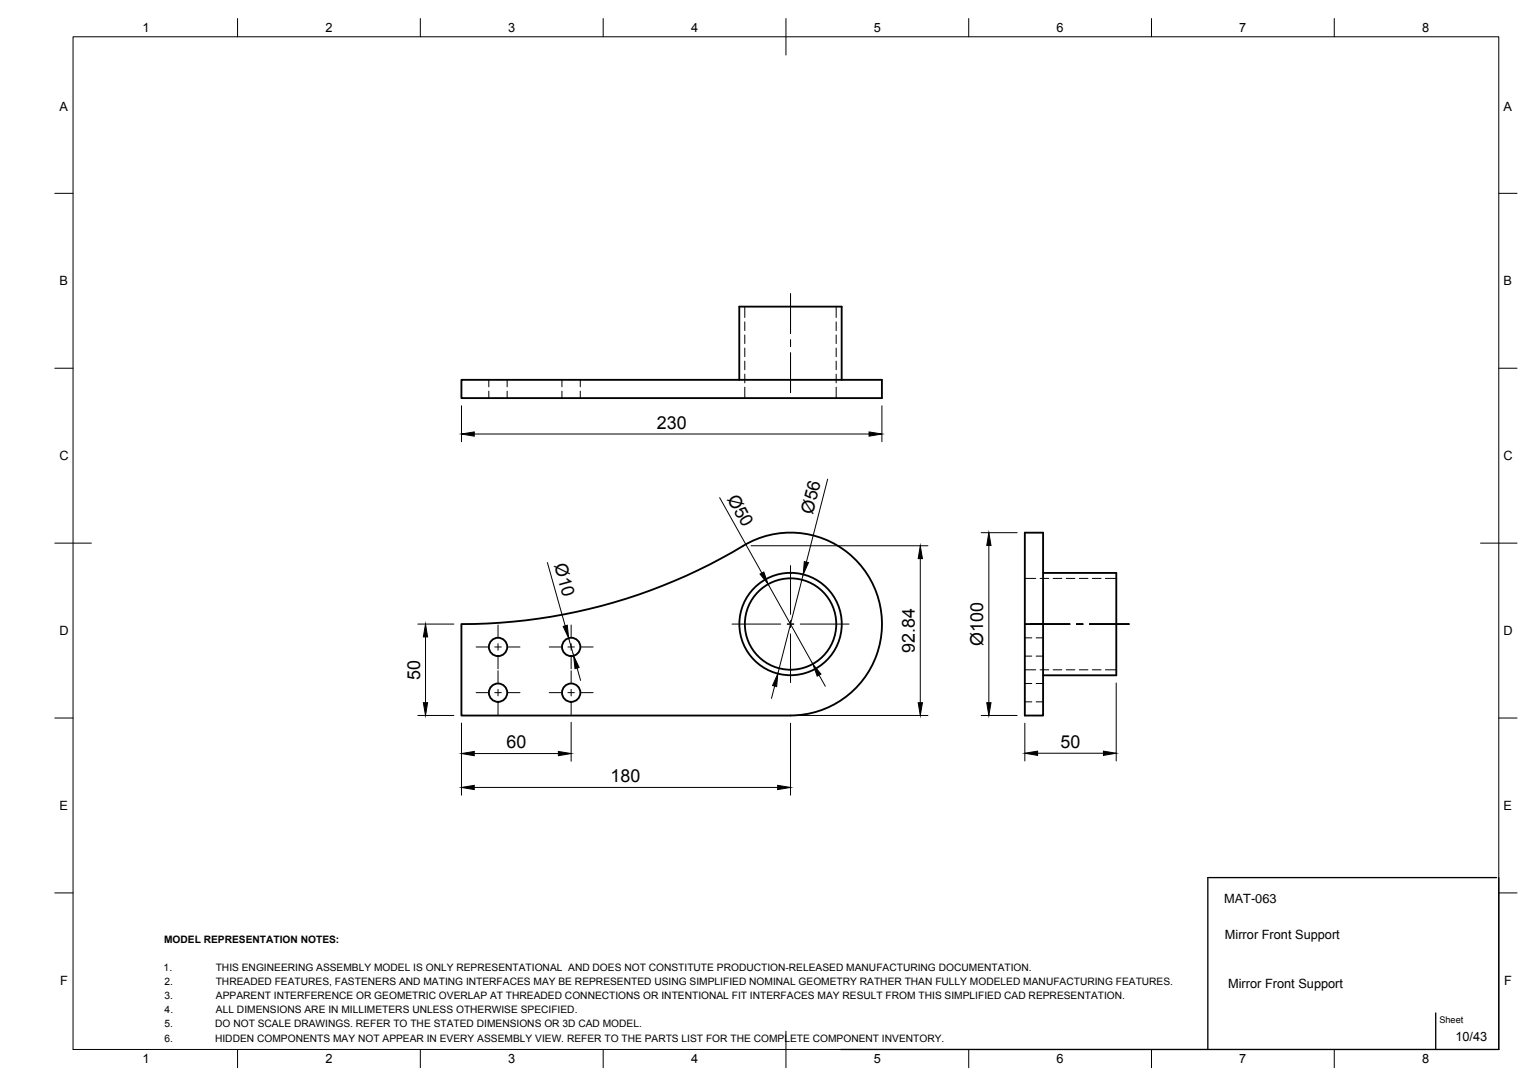
ISO-10303-21;
HEADER;
/* Generated by software containing ST-Developer
 * from STEP Tools, Inc. (www.steptools.com) 
 */

FILE_DESCRIPTION(
/* description */ (''),
/* implementation_level */ '2;1');

FILE_NAME(
/* name */ 'Mirror Front Support.step',
/* time_stamp */ '2026-10-24T09:43:01-07:00',
/* author */ (''),
/* organization */ (''),
/* preprocessor_version */ 'ST-DEVELOPER v20.2',
/* originating_system */ 'Autodesk Translation Framework v15.15.0.0',
/* authorisation */ '');

FILE_SCHEMA (('AUTOMOTIVE_DESIGN { 1 0 10303 214 3 1 1 }'));
ENDSEC;

DATA;
#10=MECHANICAL_DESIGN_GEOMETRIC_PRESENTATION_REPRESENTATION('',(#280),#11112);
#214=SHAPE_REPRESENTATION_RELATIONSHIP('SRR','None',#11237,#247);
#247=ADVANCED_BREP_SHAPE_REPRESENTATION('',(#313),#11082);
#280=STYLED_ITEM('',(#11426),#313);
#313=MANIFOLD_SOLID_BREP('Mirror Front Support',#6017);
#397=FACE_BOUND('',#1228,.T.);
#398=FACE_BOUND('',#1230,.T.);
#399=FACE_BOUND('',#1231,.T.);
#400=FACE_BOUND('',#1232,.T.);
#401=FACE_BOUND('',#1233,.T.);
#402=FACE_BOUND('',#1234,.T.);
#403=FACE_BOUND('',#1245,.T.);
#404=FACE_BOUND('',#1246,.T.);
#405=FACE_BOUND('',#1247,.T.);
#406=FACE_BOUND('',#1248,.T.);
#407=FACE_BOUND('',#1249,.T.);
#534=PLANE('',#6742);
#535=PLANE('',#6744);
#536=PLANE('',#6761);
#537=PLANE('',#6762);
#538=PLANE('',#6767);
#804=FACE_OUTER_BOUND('',#1226,.T.);
#805=FACE_OUTER_BOUND('',#1227,.T.);
#806=FACE_OUTER_BOUND('',#1229,.T.);
#807=FACE_OUTER_BOUND('',#1235,.T.);
#808=FACE_OUTER_BOUND('',#1236,.T.);
#809=FACE_OUTER_BOUND('',#1237,.T.);
#810=FACE_OUTER_BOUND('',#1238,.T.);
#811=FACE_OUTER_BOUND('',#1239,.T.);
#812=FACE_OUTER_BOUND('',#1240,.T.);
#813=FACE_OUTER_BOUND('',#1241,.T.);
#814=FACE_OUTER_BOUND('',#1242,.T.);
#815=FACE_OUTER_BOUND('',#1243,.T.);
#816=FACE_OUTER_BOUND('',#1244,.T.);
#1226=EDGE_LOOP('',(#4519,#4520,#4521,#4522));
#1227=EDGE_LOOP('',(#4523));
#1228=EDGE_LOOP('',(#4524));
#1229=EDGE_LOOP('',(#4525,#4526,#4527,#4528));
#1230=EDGE_LOOP('',(#4529));
#1231=EDGE_LOOP('',(#4530));
#1232=EDGE_LOOP('',(#4531));
#1233=EDGE_LOOP('',(#4532));
#1234=EDGE_LOOP('',(#4533));
#1235=EDGE_LOOP('',(#4534,#4535,#4536,#4537));
#1236=EDGE_LOOP('',(#4538,#4539,#4540,#4541));
#1237=EDGE_LOOP('',(#4542,#4543,#4544,#4545));
#1238=EDGE_LOOP('',(#4546,#4547,#4548,#4549));
#1239=EDGE_LOOP('',(#4550,#4551,#4552,#4553));
#1240=EDGE_LOOP('',(#4554,#4555,#4556,#4557));
#1241=EDGE_LOOP('',(#4558,#4559,#4560,#4561));
#1242=EDGE_LOOP('',(#4562,#4563,#4564,#4565));
#1243=EDGE_LOOP('',(#4566,#4567,#4568,#4569));
#1244=EDGE_LOOP('',(#4570,#4571,#4572,#4573));
#1245=EDGE_LOOP('',(#4574));
#1246=EDGE_LOOP('',(#4575));
#1247=EDGE_LOOP('',(#4576));
#1248=EDGE_LOOP('',(#4577));
#1249=EDGE_LOOP('',(#4578));
#1649=LINE('',#9930,#2008);
#1650=LINE('',#9940,#2009);
#1651=LINE('',#9942,#2010);
#1652=LINE('',#9955,#2011);
#1653=LINE('',#9959,#2012);
#1654=LINE('',#9963,#2013);
#1655=LINE('',#9967,#2014);
#1656=LINE('',#9971,#2015);
#1657=LINE('',#9974,#2016);
#1658=LINE('',#9976,#2017);
#1659=LINE('',#9977,#2018);
#1660=LINE('',#9980,#2019);
#1661=LINE('',#9981,#2020);
#1662=LINE('',#9984,#2021);
#2008=VECTOR('',#8019,0.028);
#2009=VECTOR('',#8030,0.01);
#2010=VECTOR('',#8031,0.01);
#2011=VECTOR('',#8046,0.025);
#2012=VECTOR('',#8051,0.0049999999999998);
#2013=VECTOR('',#8056,0.005);
#2014=VECTOR('',#8061,0.0049999999999998);
#2015=VECTOR('',#8066,0.005);
#2016=VECTOR('',#8069,0.01);
#2017=VECTOR('',#8070,0.01);
#2018=VECTOR('',#8071,0.01);
#2019=VECTOR('',#8074,0.01);
#2020=VECTOR('',#8075,0.01);
#2021=VECTOR('',#8078,0.01);
#2468=CIRCLE('',#6740,0.028);
#2469=CIRCLE('',#6741,0.028);
#2470=CIRCLE('',#6743,0.025);
#2471=CIRCLE('',#6745,0.299);
#2472=CIRCLE('',#6746,0.05);
#2473=CIRCLE('',#6747,0.005);
#2474=CIRCLE('',#6748,0.0049999999999998);
#2475=CIRCLE('',#6749,0.005);
#2476=CIRCLE('',#6750,0.0049999999999998);
#2477=CIRCLE('',#6752,0.025);
#2478=CIRCLE('',#6754,0.0049999999999998);
#2479=CIRCLE('',#6756,0.005);
#2480=CIRCLE('',#6758,0.0049999999999998);
#2481=CIRCLE('',#6760,0.005);
#2482=CIRCLE('',#6764,0.05);
#2483=CIRCLE('',#6766,0.299);
#2860=VERTEX_POINT('',#9927);
#2861=VERTEX_POINT('',#9929);
#2862=VERTEX_POINT('',#9933);
#2863=VERTEX_POINT('',#9936);
#2864=VERTEX_POINT('',#9937);
#2865=VERTEX_POINT('',#9939);
#2866=VERTEX_POINT('',#9941);
#2867=VERTEX_POINT('',#9944);
#2868=VERTEX_POINT('',#9946);
#2869=VERTEX_POINT('',#9948);
#2870=VERTEX_POINT('',#9950);
#2871=VERTEX_POINT('',#9953);
#2872=VERTEX_POINT('',#9957);
#2873=VERTEX_POINT('',#9961);
#2874=VERTEX_POINT('',#9965);
#2875=VERTEX_POINT('',#9969);
#2876=VERTEX_POINT('',#9973);
#2877=VERTEX_POINT('',#9975);
#2878=VERTEX_POINT('',#9979);
#2879=VERTEX_POINT('',#9983);
#3463=EDGE_CURVE('',#2860,#2860,#2468,.F.);
#3464=EDGE_CURVE('',#2860,#2861,#1649,.T.);
#3465=EDGE_CURVE('',#2861,#2861,#2469,.T.);
#3466=EDGE_CURVE('',#2862,#2862,#2470,.F.);
#3467=EDGE_CURVE('',#2863,#2864,#2471,.T.);
#3468=EDGE_CURVE('',#2865,#2863,#1650,.T.);
#3469=EDGE_CURVE('',#2866,#2865,#1651,.T.);
#3470=EDGE_CURVE('',#2864,#2866,#2472,.F.);
#3471=EDGE_CURVE('',#2867,#2867,#2473,.T.);
#3472=EDGE_CURVE('',#2868,#2868,#2474,.T.);
#3473=EDGE_CURVE('',#2869,#2869,#2475,.T.);
#3474=EDGE_CURVE('',#2870,#2870,#2476,.T.);
#3475=EDGE_CURVE('',#2871,#2871,#2477,.T.);
#3476=EDGE_CURVE('',#2871,#2862,#1652,.T.);
#3477=EDGE_CURVE('',#2872,#2872,#2478,.T.);
#3478=EDGE_CURVE('',#2872,#2870,#1653,.T.);
#3479=EDGE_CURVE('',#2873,#2873,#2479,.T.);
#3480=EDGE_CURVE('',#2873,#2869,#1654,.T.);
#3481=EDGE_CURVE('',#2874,#2874,#2480,.T.);
#3482=EDGE_CURVE('',#2874,#2868,#1655,.T.);
#3483=EDGE_CURVE('',#2875,#2875,#2481,.T.);
#3484=EDGE_CURVE('',#2875,#2867,#1656,.T.);
#3485=EDGE_CURVE('',#2865,#2876,#1657,.T.);
#3486=EDGE_CURVE('',#2877,#2863,#1658,.T.);
#3487=EDGE_CURVE('',#2876,#2877,#1659,.T.);
#3488=EDGE_CURVE('',#2876,#2878,#1660,.T.);
#3489=EDGE_CURVE('',#2878,#2866,#1661,.T.);
#3490=EDGE_CURVE('',#2879,#2864,#1662,.F.);
#3491=EDGE_CURVE('',#2878,#2879,#2482,.T.);
#3492=EDGE_CURVE('',#2877,#2879,#2483,.T.);
#4519=ORIENTED_EDGE('',*,*,#3463,.T.);
#4520=ORIENTED_EDGE('',*,*,#3464,.T.);
#4521=ORIENTED_EDGE('',*,*,#3465,.T.);
#4522=ORIENTED_EDGE('',*,*,#3464,.F.);
#4523=ORIENTED_EDGE('',*,*,#3465,.F.);
#4524=ORIENTED_EDGE('',*,*,#3466,.T.);
#4525=ORIENTED_EDGE('',*,*,#3467,.F.);
#4526=ORIENTED_EDGE('',*,*,#3468,.F.);
#4527=ORIENTED_EDGE('',*,*,#3469,.F.);
#4528=ORIENTED_EDGE('',*,*,#3470,.F.);
#4529=ORIENTED_EDGE('',*,*,#3471,.F.);
#4530=ORIENTED_EDGE('',*,*,#3472,.F.);
#4531=ORIENTED_EDGE('',*,*,#3473,.F.);
#4532=ORIENTED_EDGE('',*,*,#3474,.F.);
#4533=ORIENTED_EDGE('',*,*,#3463,.F.);
#4534=ORIENTED_EDGE('',*,*,#3475,.F.);
#4535=ORIENTED_EDGE('',*,*,#3476,.T.);
#4536=ORIENTED_EDGE('',*,*,#3466,.F.);
#4537=ORIENTED_EDGE('',*,*,#3476,.F.);
#4538=ORIENTED_EDGE('',*,*,#3477,.F.);
#4539=ORIENTED_EDGE('',*,*,#3478,.T.);
#4540=ORIENTED_EDGE('',*,*,#3474,.T.);
#4541=ORIENTED_EDGE('',*,*,#3478,.F.);
#4542=ORIENTED_EDGE('',*,*,#3479,.F.);
#4543=ORIENTED_EDGE('',*,*,#3480,.T.);
#4544=ORIENTED_EDGE('',*,*,#3473,.T.);
#4545=ORIENTED_EDGE('',*,*,#3480,.F.);
#4546=ORIENTED_EDGE('',*,*,#3481,.F.);
#4547=ORIENTED_EDGE('',*,*,#3482,.T.);
#4548=ORIENTED_EDGE('',*,*,#3472,.T.);
#4549=ORIENTED_EDGE('',*,*,#3482,.F.);
#4550=ORIENTED_EDGE('',*,*,#3483,.F.);
#4551=ORIENTED_EDGE('',*,*,#3484,.T.);
#4552=ORIENTED_EDGE('',*,*,#3471,.T.);
#4553=ORIENTED_EDGE('',*,*,#3484,.F.);
#4554=ORIENTED_EDGE('',*,*,#3485,.F.);
#4555=ORIENTED_EDGE('',*,*,#3468,.T.);
#4556=ORIENTED_EDGE('',*,*,#3486,.F.);
#4557=ORIENTED_EDGE('',*,*,#3487,.F.);
#4558=ORIENTED_EDGE('',*,*,#3469,.T.);
#4559=ORIENTED_EDGE('',*,*,#3485,.T.);
#4560=ORIENTED_EDGE('',*,*,#3488,.T.);
#4561=ORIENTED_EDGE('',*,*,#3489,.T.);
#4562=ORIENTED_EDGE('',*,*,#3490,.T.);
#4563=ORIENTED_EDGE('',*,*,#3470,.T.);
#4564=ORIENTED_EDGE('',*,*,#3489,.F.);
#4565=ORIENTED_EDGE('',*,*,#3491,.T.);
#4566=ORIENTED_EDGE('',*,*,#3467,.T.);
#4567=ORIENTED_EDGE('',*,*,#3490,.F.);
#4568=ORIENTED_EDGE('',*,*,#3492,.F.);
#4569=ORIENTED_EDGE('',*,*,#3486,.T.);
#4570=ORIENTED_EDGE('',*,*,#3487,.T.);
#4571=ORIENTED_EDGE('',*,*,#3492,.T.);
#4572=ORIENTED_EDGE('',*,*,#3491,.F.);
#4573=ORIENTED_EDGE('',*,*,#3488,.F.);
#4574=ORIENTED_EDGE('',*,*,#3483,.T.);
#4575=ORIENTED_EDGE('',*,*,#3477,.T.);
#4576=ORIENTED_EDGE('',*,*,#3479,.T.);
#4577=ORIENTED_EDGE('',*,*,#3481,.T.);
#4578=ORIENTED_EDGE('',*,*,#3475,.T.);
#5554=CYLINDRICAL_SURFACE('',#6739,0.028);
#5555=CYLINDRICAL_SURFACE('',#6751,0.025);
#5556=CYLINDRICAL_SURFACE('',#6753,0.0049999999999998);
#5557=CYLINDRICAL_SURFACE('',#6755,0.005);
#5558=CYLINDRICAL_SURFACE('',#6757,0.0049999999999998);
#5559=CYLINDRICAL_SURFACE('',#6759,0.005);
#5560=CYLINDRICAL_SURFACE('',#6763,0.05);
#5561=CYLINDRICAL_SURFACE('',#6765,0.299);
#5777=ADVANCED_FACE('',(#804),#5554,.T.);
#5778=ADVANCED_FACE('',(#805,#397),#534,.T.);
#5779=ADVANCED_FACE('',(#806,#398,#399,#400,#401,#402),#535,.F.);
#5780=ADVANCED_FACE('',(#807),#5555,.F.);
#5781=ADVANCED_FACE('',(#808),#5556,.F.);
#5782=ADVANCED_FACE('',(#809),#5557,.F.);
#5783=ADVANCED_FACE('',(#810),#5558,.F.);
#5784=ADVANCED_FACE('',(#811),#5559,.F.);
#5785=ADVANCED_FACE('',(#812),#536,.F.);
#5786=ADVANCED_FACE('',(#813),#537,.T.);
#5787=ADVANCED_FACE('',(#814),#5560,.T.);
#5788=ADVANCED_FACE('',(#815),#5561,.F.);
#5789=ADVANCED_FACE('',(#816,#403,#404,#405,#406,#407),#538,.T.);
#6017=CLOSED_SHELL('',(#5777,#5778,#5779,#5780,#5781,#5782,#5783,#5784,
#5785,#5786,#5787,#5788,#5789));
#6738=AXIS2_PLACEMENT_3D('',#9925,#8013,#8014);
#6739=AXIS2_PLACEMENT_3D('',#9926,#8015,#8016);
#6740=AXIS2_PLACEMENT_3D('',#9928,#8017,#8018);
#6741=AXIS2_PLACEMENT_3D('',#9931,#8020,#8021);
#6742=AXIS2_PLACEMENT_3D('',#9932,#8022,#8023);
#6743=AXIS2_PLACEMENT_3D('',#9934,#8024,#8025);
#6744=AXIS2_PLACEMENT_3D('',#9935,#8026,#8027);
#6745=AXIS2_PLACEMENT_3D('',#9938,#8028,#8029);
#6746=AXIS2_PLACEMENT_3D('',#9943,#8032,#8033);
#6747=AXIS2_PLACEMENT_3D('',#9945,#8034,#8035);
#6748=AXIS2_PLACEMENT_3D('',#9947,#8036,#8037);
#6749=AXIS2_PLACEMENT_3D('',#9949,#8038,#8039);
#6750=AXIS2_PLACEMENT_3D('',#9951,#8040,#8041);
#6751=AXIS2_PLACEMENT_3D('',#9952,#8042,#8043);
#6752=AXIS2_PLACEMENT_3D('',#9954,#8044,#8045);
#6753=AXIS2_PLACEMENT_3D('',#9956,#8047,#8048);
#6754=AXIS2_PLACEMENT_3D('',#9958,#8049,#8050);
#6755=AXIS2_PLACEMENT_3D('',#9960,#8052,#8053);
#6756=AXIS2_PLACEMENT_3D('',#9962,#8054,#8055);
#6757=AXIS2_PLACEMENT_3D('',#9964,#8057,#8058);
#6758=AXIS2_PLACEMENT_3D('',#9966,#8059,#8060);
#6759=AXIS2_PLACEMENT_3D('',#9968,#8062,#8063);
#6760=AXIS2_PLACEMENT_3D('',#9970,#8064,#8065);
#6761=AXIS2_PLACEMENT_3D('',#9972,#8067,#8068);
#6762=AXIS2_PLACEMENT_3D('',#9978,#8072,#8073);
#6763=AXIS2_PLACEMENT_3D('',#9982,#8076,#8077);
#6764=AXIS2_PLACEMENT_3D('',#9985,#8079,#8080);
#6765=AXIS2_PLACEMENT_3D('',#9986,#8081,#8082);
#6766=AXIS2_PLACEMENT_3D('',#9987,#8083,#8084);
#6767=AXIS2_PLACEMENT_3D('',#9988,#8085,#8086);
#8013=DIRECTION('axis',(0.,0.,1.));
#8014=DIRECTION('refdir',(1.,0.,0.));
#8015=DIRECTION('center_axis',(-1.,0.,0.));
#8016=DIRECTION('ref_axis',(0.,0.,1.));
#8017=DIRECTION('center_axis',(-1.,0.,0.));
#8018=DIRECTION('ref_axis',(0.,0.,1.));
#8019=DIRECTION('',(1.,0.,0.));
#8020=DIRECTION('center_axis',(-1.,0.,0.));
#8021=DIRECTION('ref_axis',(0.,0.,1.));
#8022=DIRECTION('center_axis',(1.,9.92686658991245E-16,-1.01959257413342E-15));
#8023=DIRECTION('ref_axis',(-1.01959257413342E-15,0.,-1.));
#8024=DIRECTION('center_axis',(1.,0.,0.));
#8025=DIRECTION('ref_axis',(0.,0.,-1.));
#8026=DIRECTION('center_axis',(-1.,0.,0.));
#8027=DIRECTION('ref_axis',(0.,0.,1.));
#8028=DIRECTION('center_axis',(1.,0.,0.));
#8029=DIRECTION('ref_axis',(0.,0.,-1.));
#8030=DIRECTION('',(0.,1.,0.));
#8031=DIRECTION('',(0.,0.,1.));
#8032=DIRECTION('center_axis',(1.,0.,0.));
#8033=DIRECTION('ref_axis',(0.,0.,-1.));
#8034=DIRECTION('center_axis',(1.,0.,0.));
#8035=DIRECTION('ref_axis',(0.,0.,-1.));
#8036=DIRECTION('center_axis',(1.,0.,0.));
#8037=DIRECTION('ref_axis',(0.,0.,-1.));
#8038=DIRECTION('center_axis',(1.,0.,0.));
#8039=DIRECTION('ref_axis',(0.,0.,-1.));
#8040=DIRECTION('center_axis',(1.,0.,0.));
#8041=DIRECTION('ref_axis',(0.,0.,-1.));
#8042=DIRECTION('center_axis',(1.,0.,0.));
#8043=DIRECTION('ref_axis',(0.,0.,-1.));
#8044=DIRECTION('center_axis',(1.,0.,0.));
#8045=DIRECTION('ref_axis',(0.,0.,-1.));
#8046=DIRECTION('',(1.,0.,0.));
#8047=DIRECTION('center_axis',(1.,0.,0.));
#8048=DIRECTION('ref_axis',(0.,0.,-1.));
#8049=DIRECTION('center_axis',(1.,0.,0.));
#8050=DIRECTION('ref_axis',(0.,0.,-1.));
#8051=DIRECTION('',(1.,0.,0.));
#8052=DIRECTION('center_axis',(1.,0.,0.));
#8053=DIRECTION('ref_axis',(0.,0.,-1.));
#8054=DIRECTION('center_axis',(1.,0.,0.));
#8055=DIRECTION('ref_axis',(0.,0.,-1.));
#8056=DIRECTION('',(1.,0.,0.));
#8057=DIRECTION('center_axis',(1.,0.,0.));
#8058=DIRECTION('ref_axis',(0.,0.,-1.));
#8059=DIRECTION('center_axis',(1.,0.,0.));
#8060=DIRECTION('ref_axis',(0.,0.,-1.));
#8061=DIRECTION('',(1.,0.,0.));
#8062=DIRECTION('center_axis',(1.,0.,0.));
#8063=DIRECTION('ref_axis',(0.,0.,-1.));
#8064=DIRECTION('center_axis',(1.,0.,0.));
#8065=DIRECTION('ref_axis',(0.,0.,-1.));
#8066=DIRECTION('',(1.,0.,0.));
#8067=DIRECTION('center_axis',(2.20458572024499E-15,-5.64627709665657E-16,
-1.));
#8068=DIRECTION('ref_axis',(-1.,8.70448729829261E-47,-2.20458572024499E-15));
#8069=DIRECTION('',(-1.,0.,0.));
#8070=DIRECTION('',(1.,0.,0.));
#8071=DIRECTION('',(0.,1.,0.));
#8072=DIRECTION('center_axis',(-3.68752647699062E-16,-1.,1.69617406532146E-17));
#8073=DIRECTION('ref_axis',(1.,-3.68752647699062E-16,0.));
#8074=DIRECTION('',(0.,0.,-1.));
#8075=DIRECTION('',(1.,0.,0.));
#8076=DIRECTION('center_axis',(1.,0.,0.));
#8077=DIRECTION('ref_axis',(0.,0.,-1.));
#8078=DIRECTION('',(-1.,0.,0.));
#8079=DIRECTION('center_axis',(1.,0.,0.));
#8080=DIRECTION('ref_axis',(0.,0.,-1.));
#8081=DIRECTION('center_axis',(1.,0.,0.));
#8082=DIRECTION('ref_axis',(0.,0.,-1.));
#8083=DIRECTION('center_axis',(1.,0.,0.));
#8084=DIRECTION('ref_axis',(0.,0.,-1.));
#8085=DIRECTION('center_axis',(-1.,0.,0.));
#8086=DIRECTION('ref_axis',(0.,0.,1.));
#9925=CARTESIAN_POINT('',(0.,0.,0.));
#9926=CARTESIAN_POINT('Origin',(-0.46,0.35,-1.1));
#9927=CARTESIAN_POINT('',(-0.5,0.35,-1.128));
#9928=CARTESIAN_POINT('Origin',(-0.5,0.35,-1.1));
#9929=CARTESIAN_POINT('',(-0.46,0.35,-1.128));
#9930=CARTESIAN_POINT('',(-0.46,0.35,-1.128));
#9931=CARTESIAN_POINT('Origin',(-0.46,0.35,-1.1));
#9932=CARTESIAN_POINT('Origin',(-0.46,0.35,-1.1));
#9933=CARTESIAN_POINT('',(-0.46,0.35,-1.075));
#9934=CARTESIAN_POINT('Origin',(-0.46,0.35,-1.1));
#9935=CARTESIAN_POINT('Origin',(-0.5,0.35003431001795,-1.0350379192153));
#9936=CARTESIAN_POINT('',(-0.500000000000482,0.35,-0.920000000000262));
#9937=CARTESIAN_POINT('',(-0.500000000000482,0.392836676218822,-1.07421203438571));
#9938=CARTESIAN_POINT('Origin',(-0.5,0.649,-0.92));
#9939=CARTESIAN_POINT('',(-0.5,0.3,-0.92));
#9940=CARTESIAN_POINT('',(-0.5,0.3,-0.92));
#9941=CARTESIAN_POINT('',(-0.5,0.3,-1.09999999999836));
#9942=CARTESIAN_POINT('',(-0.5,0.3,-1.09999999952063));
#9943=CARTESIAN_POINT('Origin',(-0.5,0.35,-1.1));
#9944=CARTESIAN_POINT('',(-0.5,0.3125,-0.975));
#9945=CARTESIAN_POINT('Origin',(-0.5,0.3125,-0.98));
#9946=CARTESIAN_POINT('',(-0.5,0.3375,-0.935));
#9947=CARTESIAN_POINT('Origin',(-0.5,0.3375,-0.94));
#9948=CARTESIAN_POINT('',(-0.5,0.3375,-0.975));
#9949=CARTESIAN_POINT('Origin',(-0.5,0.3375,-0.98));
#9950=CARTESIAN_POINT('',(-0.5,0.3125,-0.935));
#9951=CARTESIAN_POINT('Origin',(-0.5,0.3125,-0.94));
#9952=CARTESIAN_POINT('Origin',(-0.51,0.35,-1.1));
#9953=CARTESIAN_POINT('',(-0.51,0.35,-1.075));
#9954=CARTESIAN_POINT('Origin',(-0.51,0.35,-1.1));
#9955=CARTESIAN_POINT('',(-0.51,0.35,-1.075));
#9956=CARTESIAN_POINT('Origin',(-0.51,0.3125,-0.94));
#9957=CARTESIAN_POINT('',(-0.51,0.3125,-0.935));
#9958=CARTESIAN_POINT('Origin',(-0.51,0.3125,-0.94));
#9959=CARTESIAN_POINT('',(-0.51,0.3125,-0.935));
#9960=CARTESIAN_POINT('Origin',(-0.51,0.3375,-0.98));
#9961=CARTESIAN_POINT('',(-0.51,0.3375,-0.975));
#9962=CARTESIAN_POINT('Origin',(-0.51,0.3375,-0.98));
#9963=CARTESIAN_POINT('',(-0.51,0.3375,-0.975));
#9964=CARTESIAN_POINT('Origin',(-0.51,0.3375,-0.94));
#9965=CARTESIAN_POINT('',(-0.51,0.3375,-0.935));
#9966=CARTESIAN_POINT('Origin',(-0.51,0.3375,-0.94));
#9967=CARTESIAN_POINT('',(-0.51,0.3375,-0.935));
#9968=CARTESIAN_POINT('Origin',(-0.51,0.3125,-0.98));
#9969=CARTESIAN_POINT('',(-0.51,0.3125,-0.975));
#9970=CARTESIAN_POINT('Origin',(-0.51,0.3125,-0.98));
#9971=CARTESIAN_POINT('',(-0.51,0.3125,-0.975));
#9972=CARTESIAN_POINT('Origin',(-0.505,0.325,-0.92));
#9973=CARTESIAN_POINT('',(-0.51,0.3,-0.92));
#9974=CARTESIAN_POINT('',(-0.500000000000001,0.3,-0.92));
#9975=CARTESIAN_POINT('',(-0.509999999999358,0.35,-0.92));
#9976=CARTESIAN_POINT('',(-0.50999999975,0.35,-0.92));
#9977=CARTESIAN_POINT('',(-0.510000000000001,0.3,-0.92));
#9978=CARTESIAN_POINT('Origin',(-0.505,0.3,-1.01));
#9979=CARTESIAN_POINT('',(-0.51,0.3,-1.09999999999807));
#9980=CARTESIAN_POINT('',(-0.510000000000001,0.3,-0.920000000000001));
#9981=CARTESIAN_POINT('',(-0.510000000000001,0.3,-1.1));
#9982=CARTESIAN_POINT('Origin',(-0.51,0.35,-1.1));
#9983=CARTESIAN_POINT('',(-0.51,0.39283667622015,-1.07421203438792));
#9984=CARTESIAN_POINT('',(-0.50000000025,0.392836676219352,-1.07421203438659));
#9985=CARTESIAN_POINT('Origin',(-0.51,0.35,-1.1));
#9986=CARTESIAN_POINT('Origin',(-0.51,0.649,-0.92));
#9987=CARTESIAN_POINT('Origin',(-0.51,0.649,-0.92));
#9988=CARTESIAN_POINT('Origin',(-0.51,0.35003431001795,-1.0350379192153));
#11043=UNCERTAINTY_MEASURE_WITH_UNIT(LENGTH_MEASURE(1.E-5),#11113,
'DISTANCE_ACCURACY_VALUE',
'Maximum model space distance between geometric entities at asserted c
onnectivities');
#11073=UNCERTAINTY_MEASURE_WITH_UNIT(LENGTH_MEASURE(1.E-5),#11113,
'DISTANCE_ACCURACY_VALUE',
'Maximum model space distance between geometric entities at asserted c
onnectivities');
#11082=(
GEOMETRIC_REPRESENTATION_CONTEXT(3)
GLOBAL_UNCERTAINTY_ASSIGNED_CONTEXT((#11043))
GLOBAL_UNIT_ASSIGNED_CONTEXT((#11113,#11114,#11115))
REPRESENTATION_CONTEXT('','3D')
);
#11112=(
GEOMETRIC_REPRESENTATION_CONTEXT(3)
GLOBAL_UNCERTAINTY_ASSIGNED_CONTEXT((#11073))
GLOBAL_UNIT_ASSIGNED_CONTEXT((#11113,#11114,#11115))
REPRESENTATION_CONTEXT('','3D')
);
#11113=(
LENGTH_UNIT()
NAMED_UNIT(*)
SI_UNIT($,.METRE.)
);
#11114=(
NAMED_UNIT(*)
PLANE_ANGLE_UNIT()
SI_UNIT($,.RADIAN.)
);
#11115=(
NAMED_UNIT(*)
SI_UNIT($,.STERADIAN.)
SOLID_ANGLE_UNIT()
);
#11124=SHAPE_DEFINITION_REPRESENTATION(#11162,#11237);
#11162=PRODUCT_DEFINITION_SHAPE('',$,#11276);
#11237=SHAPE_REPRESENTATION('',(#6738),#11082);
#11267=PRODUCT_DEFINITION_CONTEXT('part definition',#11383,'design');
#11276=PRODUCT_DEFINITION('Mirror Front Support','Mirror Front Support',
#11314,#11267);
#11314=PRODUCT_DEFINITION_FORMATION('',$,#11393);
#11383=APPLICATION_CONTEXT(
'Core Data for Automotive Mechanical Design Process');
#11384=PRODUCT_CONTEXT('part definition',#11383,'mechanical');
#11393=PRODUCT('Mirror Front Support','Mirror Front Support',
'Mirrorfront_sup__ DE     8799',(#11384));
#11426=PRESENTATION_STYLE_ASSIGNMENT((#11430));
#11430=SURFACE_STYLE_USAGE(.BOTH.,#11434);
#11434=SURFACE_SIDE_STYLE('',(#11438));
#11438=SURFACE_STYLE_FILL_AREA(#11442);
#11442=FILL_AREA_STYLE('Opaque(202,209,238)',(#11446));
#11446=FILL_AREA_STYLE_COLOUR('Opaque(202,209,238)',#11450);
#11450=COLOUR_RGB('Opaque(202,209,238)',0.792156862745098,0.819607843137255,
0.933333333333333);
ENDSEC;
END-ISO-10303-21;
